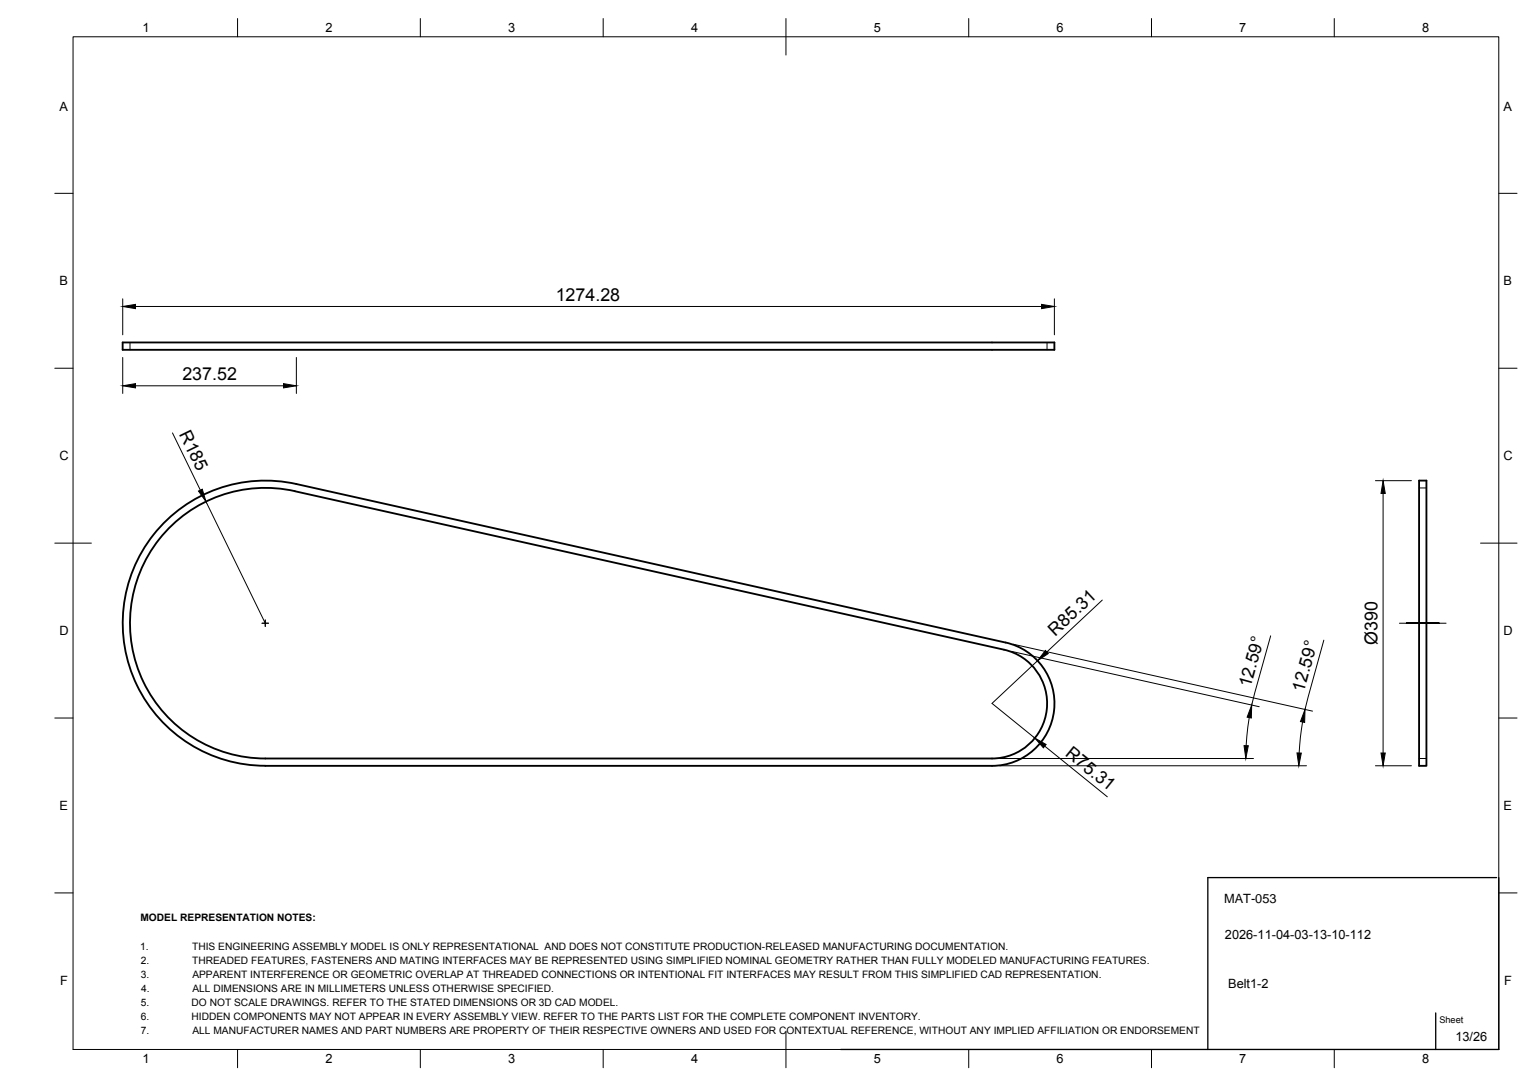
ISO-10303-21;
HEADER;
FILE_DESCRIPTION (('STEP AP214'),
    '1' );
FILE_NAME ('Belt1-2.step',
    '2026-10-10T03:43:58',
    ( '' ),
    ( '' ),
    'SwSTEP 2.0',
    'SolidWorks 2026',
    '' );
FILE_SCHEMA (( 'AUTOMOTIVE_DESIGN' ));
ENDSEC;

DATA;
#50=ORIENTED_EDGE ( 'NONE', *, *, #39637, .T. ) ;
#400=LINE ( 'NONE', #38040, #43022 ) ;
#483=ADVANCED_BREP_SHAPE_REPRESENTATION ( '', ( #63157, #66832 ), #16381 ) ;
#518=CIRCLE ( 'NONE', #7308, 85.31295361348101380 ) ;
#529=CARTESIAN_POINT ( 'NONE',  ( -737.6000277536880958, -694.2189502691660437, 10.00000000000000000 ) ) ;
#744=CARTESIAN_POINT ( 'NONE',  ( -783.0172411895269988, -622.0000000000060254, 0.000000000000000000 ) ) ;
#772=VERTEX_POINT ( 'NONE', #33537 ) ;
#796=CARTESIAN_POINT ( 'NONE',  ( -783.0172411895269988, -622.0000000000060254, 10.00000000000000000 ) ) ;
#912=( GEOMETRIC_REPRESENTATION_CONTEXT ( 3 ) GLOBAL_UNCERTAINTY_ASSIGNED_CONTEXT ( ( #67666 ) ) GLOBAL_UNIT_ASSIGNED_CONTEXT ( ( #33451, #27807, #26433 ) ) REPRESENTATION_CONTEXT ( 'NONE', 'WORKASPACE' ) );
#1644=ADVANCED_FACE ( 'NONE', ( #6203 ), #36842, .F. ) ;
#1813=ORIENTED_EDGE ( 'NONE', *, *, #39226, .T. ) ;
#1988=MECHANICAL_DESIGN_GEOMETRIC_PRESENTATION_REPRESENTATION('',(#14333),#912);
#2075=VECTOR ( 'NONE', #8776, 1000.000000000000227 ) ;
#2171=VERTEX_POINT ( 'NONE', #48575 ) ;
#2420=DIRECTION ( 'NONE',  ( 0.000000000000000000, 0.000000000000000000, 1.000000000000000000 ) ) ;
#2612=CARTESIAN_POINT ( 'NONE',  ( -137.3060924980642596, 138.4631249211268482, 10.00000000000000000 ) ) ;
#2773=ORIENTED_EDGE ( 'NONE', *, *, #39637, .F. ) ;
#3415=EDGE_CURVE ( 'NONE', #35337, #45327, #38767, .T. ) ;
#4052=EDGE_LOOP ( 'NONE', ( #25158, #36833, #15279, #17366 ) ) ;
#4364=VERTEX_POINT ( 'NONE', #44294 ) ;
#4376=CYLINDRICAL_SURFACE ( 'NONE', #64379, 185.0000000000000000 ) ;
#4633=CARTESIAN_POINT ( 'NONE',  ( -843.0889760620008246, -561.4220607509099636, 0.000000000000000000 ) ) ;
#4659=ORIENTED_EDGE ( 'NONE', *, *, #47648, .T. ) ;
#4808=DIRECTION ( 'NONE',  ( -1.000000000000000000, 0.000000000000000000, 0.000000000000000000 ) ) ;
#4817=EDGE_CURVE ( 'NONE', #23974, #44398, #13439, .T. ) ;
#5033=AXIS2_PLACEMENT_3D ( 'NONE', #67529, #67881, #9476 ) ;
#5314=SURFACE_SIDE_STYLE ('',( #53485 ) ) ;
#5328=COLOUR_RGB ( '',0.7921568627450980005, 0.8196078431372548767, 0.9333333333333333481 ) ;
#5721=CARTESIAN_POINT ( 'NONE',  ( -3.841371665203041630E-11, 0.000000000000000000, 10.00000000000000000 ) ) ;
#6203=FACE_OUTER_BOUND ( 'NONE', #4052, .T. ) ;
#6217=CARTESIAN_POINT ( 'NONE',  ( -783.0172411895269988, -622.0000000000060254, 10.00000000000000000 ) ) ;
#6235=AXIS2_PLACEMENT_3D ( 'NONE', #796, #54594, #6418 ) ;
#6350=FACE_OUTER_BOUND ( 'NONE', #25484, .T. ) ;
#6353=FILL_AREA_STYLE_COLOUR ( '', #5328 ) ;
#6418=DIRECTION ( 'NONE',  ( -1.000000000000000000, 0.000000000000000000, 0.000000000000000000 ) ) ;
#6578=EDGE_CURVE ( 'NONE', #4364, #56202, #63506, .T. ) ;
#6741=EDGE_CURVE ( 'NONE', #2171, #45327, #32909, .T. ) ;
#7096=AXIS2_PLACEMENT_3D ( 'NONE', #32587, #11821, #54011 ) ;
#7308=AXIS2_PLACEMENT_3D ( 'NONE', #55891, #7709, #49903 ) ;
#7350=FACE_OUTER_BOUND ( 'NONE', #64510, .T. ) ;
#7700=CYLINDRICAL_SURFACE ( 'NONE', #43072, 75.31295361348099959 ) ;
#7709=DIRECTION ( 'NONE',  ( 0.000000000000000000, 0.000000000000000000, 1.000000000000000000 ) ) ;
#7878=CARTESIAN_POINT ( 'NONE',  ( -3.841371665203041630E-11, 0.000000000000000000, 10.00000000000000000 ) ) ;
#7930=ORIENTED_EDGE ( 'NONE', *, *, #15029, .T. ) ;
#8319=DIRECTION ( 'NONE',  ( 1.000000000000000000, 0.000000000000000000, 0.000000000000000000 ) ) ;
#8395=DIRECTION ( 'NONE',  ( 1.000000000000000000, 0.000000000000000000, 0.000000000000000000 ) ) ;
#8400=CARTESIAN_POINT ( 'NONE',  ( -836.0476379851789943, -568.5227338237882577, 10.00000000000000000 ) ) ;
#8476=APPLICATION_CONTEXT ( 'automotive_design' ) ;
#8776=DIRECTION ( 'NONE',  ( 0.8465179929926601732, 0.5323601107705934199, 0.000000000000000000 ) ) ;
#8933=LINE ( 'NONE', #2612, #15335 ) ;
#8944=CARTESIAN_POINT ( 'NONE',  ( -783.0172411895269988, -622.0000000000060254, 10.00000000000000000 ) ) ;
#8997=VERTEX_POINT ( 'NONE', #19721 ) ;
#9476=DIRECTION ( 'NONE',  ( 1.000000000000000000, 0.000000000000000000, 0.000000000000000000 ) ) ;
#9556=CIRCLE ( 'NONE', #17419, 85.31295361348101380 ) ;
#10144=VECTOR ( 'NONE', #29624, 1000.000000000000000 ) ;
#10284=( LENGTH_UNIT ( ) NAMED_UNIT ( * ) SI_UNIT ( .MILLI., .METRE. ) );
#10312=DIRECTION ( 'NONE',  ( 1.000000000000000000, 0.000000000000000000, 0.000000000000000000 ) ) ;
#10925=EDGE_CURVE ( 'NONE', #23974, #31182, #64895, .T. ) ;
#10935=AXIS2_PLACEMENT_3D ( 'NONE', #21876, #32787, #32098 ) ;
#10980=CIRCLE ( 'NONE', #18831, 185.0000000000000000 ) ;
#11158=CARTESIAN_POINT ( 'NONE',  ( -836.0476379851789943, -568.5227338237882577, 10.00000000000000000 ) ) ;
#11197=VECTOR ( 'NONE', #34857, 1000.000000000000000 ) ;
#11821=DIRECTION ( 'NONE',  ( 0.000000000000000000, 0.000000000000000000, 1.000000000000000000 ) ) ;
#11932=CARTESIAN_POINT ( 'NONE',  ( 98.48662049252135375, -156.6058287036421461, 0.000000000000000000 ) ) ;
#11981=PRESENTATION_STYLE_ASSIGNMENT (( #60160 ) ) ;
#12058=APPLICATION_CONTEXT ( 'automotive_design' ) ;
#12469=ADVANCED_FACE ( 'NONE', ( #39879, #61340 ), #34625, .T. ) ;
#12980=CARTESIAN_POINT ( 'NONE',  ( -3.841371665203041630E-11, 0.000000000000000000, 10.00000000000000000 ) ) ;
#13197=CARTESIAN_POINT ( 'NONE',  ( -3.841371665203041630E-11, 0.000000000000000000, 10.00000000000000000 ) ) ;
#13360=CARTESIAN_POINT ( 'NONE',  ( -836.0476379851791080, -568.5227338237882577, 0.000000000000000000 ) ) ;
#13395=LINE ( 'NONE', #65470, #11197 ) ;
#13439=LINE ( 'NONE', #24692, #66682 ) ;
#13783=CIRCLE ( 'NONE', #16031, 75.31295361348099959 ) ;
#13838=DIRECTION ( 'NONE',  ( 1.000000000000000000, 0.000000000000000000, 0.000000000000000000 ) ) ;
#13899=CARTESIAN_POINT ( 'NONE',  ( -137.3060924980642596, 138.4631249211268482, 10.00000000000000000 ) ) ;
#14167=DIRECTION ( 'NONE',  ( 0.7041338076821838099, -0.7100673072878298520, 0.000000000000000000 ) ) ;
#14220=DIRECTION ( 'NONE',  ( -0.000000000000000000, -0.000000000000000000, -1.000000000000000000 ) ) ;
#14333=STYLED_ITEM ( 'NONE', ( #11981 ), #63157 ) ;
#14567=ORIENTED_EDGE ( 'NONE', *, *, #47164, .F. ) ;
#15029=EDGE_CURVE ( 'NONE', #51895, #35337, #62898, .T. ) ;
#15261=ORIENTED_EDGE ( 'NONE', *, *, #6578, .T. ) ;
#15279=ORIENTED_EDGE ( 'NONE', *, *, #15029, .F. ) ;
#15319=CARTESIAN_POINT ( 'NONE',  ( 98.48662049252135375, -156.6058287036421461, 10.00000000000000000 ) ) ;
#15335=VECTOR ( 'NONE', #18788, 1000.000000000000000 ) ;
#15471=ORIENTED_EDGE ( 'NONE', *, *, #37409, .F. ) ;
#15651=EDGE_CURVE ( 'NONE', #772, #4364, #61653, .T. ) ;
#15918=SHAPE_REPRESENTATION_RELATIONSHIP ( 'NONE' , 'NONE' ,  #46431, #483 ) ;
#15964=ORIENTED_EDGE ( 'NONE', *, *, #53374, .F. ) ;
#16014=ADVANCED_FACE ( 'NONE', ( #69170 ), #20998, .T. ) ;
#16031=AXIS2_PLACEMENT_3D ( 'NONE', #6217, #49820, #44190 ) ;
#16080=ORIENTED_EDGE ( 'NONE', *, *, #39226, .F. ) ;
#16381=( GEOMETRIC_REPRESENTATION_CONTEXT ( 3 ) GLOBAL_UNCERTAINTY_ASSIGNED_CONTEXT ( ( #49374 ) ) GLOBAL_UNIT_ASSIGNED_CONTEXT ( ( #10284, #38062, #27503 ) ) REPRESENTATION_CONTEXT ( 'NONE', 'WORKASPACE' ) );
#16466=ORIENTED_EDGE ( 'NONE', *, *, #59378, .F. ) ;
#16966=EDGE_CURVE ( 'NONE', #27319, #8997, #51411, .T. ) ;
#17366=ORIENTED_EDGE ( 'NONE', *, *, #60571, .T. ) ;
#17419=AXIS2_PLACEMENT_3D ( 'NONE', #744, #37673, #22198 ) ;
#17544=ORIENTED_EDGE ( 'NONE', *, *, #62686, .T. ) ;
#17563=LINE ( 'NONE', #65769, #42289 ) ;
#17823=LINE ( 'NONE', #61074, #45554 ) ;
#18035=ADVANCED_FACE ( 'NONE', ( #42232, #64032 ), #36959, .F. ) ;
#18131=LINE ( 'NONE', #35347, #47991 ) ;
#18788=DIRECTION ( 'NONE',  ( -0.000000000000000000, -0.000000000000000000, -1.000000000000000000 ) ) ;
#18820=ADVANCED_FACE ( 'NONE', ( #62405 ), #40948, .T. ) ;
#18831=AXIS2_PLACEMENT_3D ( 'NONE', #13197, #44497, #22692 ) ;
#18943=DIRECTION ( 'NONE',  ( -1.000000000000000000, 0.000000000000000000, 0.000000000000000000 ) ) ;
#19320=CLOSED_SHELL ( 'NONE', ( #40021, #16014, #12469, #18035, #28178, #1644, #18820, #20155, #25382, #30202, #67285, #52018 ) ) ;
#19721=CARTESIAN_POINT ( 'NONE',  ( -858.3301948030079984, -622.0000000000060254, 10.00000000000000000 ) ) ;
#20155=ADVANCED_FACE ( 'NONE', ( #6350 ), #27803, .F. ) ;
#20497=FACE_OUTER_BOUND ( 'NONE', #36320, .T. ) ;
#20652=CARTESIAN_POINT ( 'NONE',  ( -137.3060924980642596, 138.4631249211268482, 10.00000000000000000 ) ) ;
#20687=ORIENTED_EDGE ( 'NONE', *, *, #34883, .T. ) ;
#20771=CARTESIAN_POINT ( 'NONE',  ( -3.841371665203041630E-11, 0.000000000000000000, 0.000000000000000000 ) ) ;
#20998=CYLINDRICAL_SURFACE ( 'NONE', #65260, 85.31295361348101380 ) ;
#21143=ORIENTED_EDGE ( 'NONE', *, *, #47164, .T. ) ;
#21789=AXIS2_PLACEMENT_3D ( 'NONE', #25794, #31408, #13838 ) ;
#21825=FILL_AREA_STYLE ('',( #6353 ) ) ;
#21876=CARTESIAN_POINT ( 'NONE',  ( 98.48662049252141060, -156.6058287036421177, 10.00000000000000000 ) ) ;
#22198=DIRECTION ( 'NONE',  ( 1.000000000000000000, 0.000000000000000000, 0.000000000000000000 ) ) ;
#22214=DIRECTION ( 'NONE',  ( -0.000000000000000000, -0.000000000000000000, -1.000000000000000000 ) ) ;
#22249=FACE_OUTER_BOUND ( 'NONE', #61024, .T. ) ;
#22256=LINE ( 'NONE', #48960, #40432 ) ;
#22692=DIRECTION ( 'NONE',  ( 1.000000000000000000, 0.000000000000000000, 0.000000000000000000 ) ) ;
#23210=ORIENTED_EDGE ( 'NONE', *, *, #50303, .F. ) ;
#23231=ORIENTED_EDGE ( 'NONE', *, *, #6578, .F. ) ;
#23502=FACE_OUTER_BOUND ( 'NONE', #52077, .T. ) ;
#23851=CARTESIAN_POINT ( 'NONE',  ( -3.841371665203041630E-11, 0.000000000000000000, 10.00000000000000000 ) ) ;
#23972=CIRCLE ( 'NONE', #7096, 185.0000000000000000 ) ;
#23974=VERTEX_POINT ( 'NONE', #29767 ) ;
#24090=DIRECTION ( 'NONE',  ( -1.000000000000000000, 0.000000000000000000, 0.000000000000000000 ) ) ;
#24259=CARTESIAN_POINT ( 'NONE',  ( -737.6000277536880958, -694.2189502691659300, 10.00000000000000000 ) ) ;
#24630=DIRECTION ( 'NONE',  ( -0.8465179929926601732, -0.5323601107705934199, 0.000000000000000000 ) ) ;
#24692=CARTESIAN_POINT ( 'NONE',  ( -868.3301948030079984, -622.0000000000060254, 10.00000000000000000 ) ) ;
#24825=EDGE_LOOP ( 'NONE', ( #4659, #54553, #25083, #1813, #17544 ) ) ;
#25083=ORIENTED_EDGE ( 'NONE', *, *, #59378, .T. ) ;
#25158=ORIENTED_EDGE ( 'NONE', *, *, #6741, .T. ) ;
#25382=ADVANCED_FACE ( 'NONE', ( #22249 ), #65162, .F. ) ;
#25383=PRODUCT ( 'Belt1-2', 'Belt1-2', '', ( #62124 ) ) ;
#25484=EDGE_LOOP ( 'NONE', ( #39915, #52107, #61469, #50 ) ) ;
#25591=AXIS2_PLACEMENT_3D ( 'NONE', #7878, #29328, #34144 ) ;
#25794=CARTESIAN_POINT ( 'NONE',  ( -3.841371665203041630E-11, 0.000000000000000000, 0.000000000000000000 ) ) ;
#26049=AXIS2_PLACEMENT_3D ( 'NONE', #20771, #32027, #65071 ) ;
#26141=EDGE_CURVE ( 'NONE', #45146, #51895, #60214, .T. ) ;
#26226=SHAPE_DEFINITION_REPRESENTATION ( #30409, #46431 ) ;
#26433=( NAMED_UNIT ( * ) SI_UNIT ( $, .STERADIAN. ) SOLID_ANGLE_UNIT ( ) );
#26631=DIRECTION ( 'NONE',  ( 0.7041338076821838099, -0.7100673072878299630, 0.000000000000000000 ) ) ;
#26818=EDGE_CURVE ( 'NONE', #44398, #46298, #9556, .T. ) ;
#27319=VERTEX_POINT ( 'NONE', #28624 ) ;
#27327=VECTOR ( 'NONE', #54051, 1000.000000000000000 ) ;
#27445=VERTEX_POINT ( 'NONE', #57433 ) ;
#27503=( NAMED_UNIT ( * ) SI_UNIT ( $, .STERADIAN. ) SOLID_ANGLE_UNIT ( ) );
#27615=AXIS2_PLACEMENT_3D ( 'NONE', #12980, #39355, #18943 ) ;
#27632=CARTESIAN_POINT ( 'NONE',  ( -137.3060924980642596, 138.4631249211268482, 0.000000000000000000 ) ) ;
#27803=PLANE ( 'NONE',  #28332 ) ;
#27807=( NAMED_UNIT ( * ) PLANE_ANGLE_UNIT ( ) SI_UNIT ( $, .RADIAN. ) );
#28178=ADVANCED_FACE ( 'NONE', ( #51648 ), #45320, .T. ) ;
#28332=AXIS2_PLACEMENT_3D ( 'NONE', #49243, #29894, #24630 ) ;
#28472=ORIENTED_EDGE ( 'NONE', *, *, #6741, .F. ) ;
#28624=CARTESIAN_POINT ( 'NONE',  ( -836.0476379851789943, -568.5227338237882577, 10.00000000000000000 ) ) ;
#29153=EDGE_CURVE ( 'NONE', #45146, #58415, #17563, .T. ) ;
#29328=DIRECTION ( 'NONE',  ( 0.000000000000000000, 0.000000000000000000, 1.000000000000000000 ) ) ;
#29344=ORIENTED_EDGE ( 'NONE', *, *, #69178, .T. ) ;
#29624=DIRECTION ( 'NONE',  ( -0.000000000000000000, -0.000000000000000000, -1.000000000000000000 ) ) ;
#29767=CARTESIAN_POINT ( 'NONE',  ( -868.3301948030079984, -622.0000000000060254, 10.00000000000000000 ) ) ;
#29894=DIRECTION ( 'NONE',  ( -0.5323601107705935309, 0.8465179929926602842, 0.000000000000000000 ) ) ;
#30201=DIRECTION ( 'NONE',  ( -0.7100673072878298520, -0.7041338076821836989, 0.000000000000000000 ) ) ;
#30202=ADVANCED_FACE ( 'NONE', ( #20497 ), #59160, .T. ) ;
#30409=PRODUCT_DEFINITION_SHAPE ( 'NONE', 'NONE',  #54682 ) ;
#30539=CARTESIAN_POINT ( 'NONE',  ( -137.3060924980642596, 138.4631249211268482, 10.00000000000000000 ) ) ;
#31087=CARTESIAN_POINT ( 'NONE',  ( -742.9236288613935812, -685.7537703392392814, 10.00000000000000000 ) ) ;
#31182=VERTEX_POINT ( 'NONE', #529 ) ;
#31408=DIRECTION ( 'NONE',  ( 0.000000000000000000, 0.000000000000000000, 1.000000000000000000 ) ) ;
#31420=ORIENTED_EDGE ( 'NONE', *, *, #16966, .T. ) ;
#32016=VECTOR ( 'NONE', #57545, 1000.000000000000000 ) ;
#32027=DIRECTION ( 'NONE',  ( 0.000000000000000000, 0.000000000000000000, 1.000000000000000000 ) ) ;
#32098=DIRECTION ( 'NONE',  ( -0.8465179929926601732, -0.5323601107705934199, 0.000000000000000000 ) ) ;
#32587=CARTESIAN_POINT ( 'NONE',  ( -3.841371665203041630E-11, 0.000000000000000000, 0.000000000000000000 ) ) ;
#32648=ORIENTED_EDGE ( 'NONE', *, *, #56944, .F. ) ;
#32695=DIRECTION ( 'NONE',  ( -0.000000000000000000, -0.000000000000000000, -1.000000000000000000 ) ) ;
#32702=ORIENTED_EDGE ( 'NONE', *, *, #69229, .T. ) ;
#32787=DIRECTION ( 'NONE',  ( -0.5323601107705935309, 0.8465179929926602842, 0.000000000000000000 ) ) ;
#32812=ORIENTED_EDGE ( 'NONE', *, *, #50303, .T. ) ;
#32909=LINE ( 'NONE', #27632, #33121 ) ;
#32935=DIRECTION ( 'NONE',  ( 0.7100673072878298520, 0.7041338076821836989, 0.000000000000000000 ) ) ;
#33121=VECTOR ( 'NONE', #49069, 1000.000000000000114 ) ;
#33204=EDGE_LOOP ( 'NONE', ( #49834, #56468, #51894, #56685, #28472 ) ) ;
#33451=( LENGTH_UNIT ( ) NAMED_UNIT ( * ) SI_UNIT ( .MILLI., .METRE. ) );
#33537=CARTESIAN_POINT ( 'NONE',  ( -742.9236288613935812, -685.7537703392392814, 10.00000000000000000 ) ) ;
#34133=ORIENTED_EDGE ( 'NONE', *, *, #69229, .F. ) ;
#34144=DIRECTION ( 'NONE',  ( 1.000000000000000000, 0.000000000000000000, -0.000000000000000000 ) ) ;
#34194=DIRECTION ( 'NONE',  ( -0.000000000000000000, -0.000000000000000000, -1.000000000000000000 ) ) ;
#34218=ORIENTED_EDGE ( 'NONE', *, *, #10925, .T. ) ;
#34226=VECTOR ( 'NONE', #40058, 1000.000000000000227 ) ;
#34568=ORIENTED_EDGE ( 'NONE', *, *, #4817, .F. ) ;
#34584=CARTESIAN_POINT ( 'NONE',  ( -130.2647544212423725, 131.3624518482485541, 10.00000000000000000 ) ) ;
#34625=PLANE ( 'NONE',  #25591 ) ;
#34857=DIRECTION ( 'NONE',  ( -0.000000000000000000, -0.000000000000000000, -1.000000000000000000 ) ) ;
#34883=EDGE_CURVE ( 'NONE', #8997, #64350, #13395, .T. ) ;
#34930=CARTESIAN_POINT ( 'NONE',  ( 98.48662049252141060, -156.6058287036421177, 10.00000000000000000 ) ) ;
#35109=DIRECTION ( 'NONE',  ( -0.000000000000000000, -0.000000000000000000, -1.000000000000000000 ) ) ;
#35173=CARTESIAN_POINT ( 'NONE',  ( -868.3301948030079984, -622.0000000000060254, 0.000000000000000000 ) ) ;
#35276=CARTESIAN_POINT ( 'NONE',  ( -836.0476379851789943, -568.5227338237882577, 10.00000000000000000 ) ) ;
#35337=VERTEX_POINT ( 'NONE', #68499 ) ;
#35347=CARTESIAN_POINT ( 'NONE',  ( -836.0476379851789943, -568.5227338237882577, 0.000000000000000000 ) ) ;
#36292=EDGE_LOOP ( 'NONE', ( #42354, #7930, #21143, #34218, #55338 ) ) ;
#36320=EDGE_LOOP ( 'NONE', ( #16466, #15471, #55287, #15261 ) ) ;
#36486=CARTESIAN_POINT ( 'NONE',  ( -783.0172411895269988, -622.0000000000060254, 10.00000000000000000 ) ) ;
#36487=DIRECTION ( 'NONE',  ( 1.000000000000000000, 0.000000000000000000, 0.000000000000000000 ) ) ;
#36833=ORIENTED_EDGE ( 'NONE', *, *, #3415, .F. ) ;
#36842=PLANE ( 'NONE',  #58757 ) ;
#36959=PLANE ( 'NONE',  #26049 ) ;
#37409=EDGE_CURVE ( 'NONE', #772, #54998, #53195, .T. ) ;
#37673=DIRECTION ( 'NONE',  ( 0.000000000000000000, 0.000000000000000000, 1.000000000000000000 ) ) ;
#38040=CARTESIAN_POINT ( 'NONE',  ( -737.6000277536880958, -694.2189502691660437, 10.00000000000000000 ) ) ;
#38062=( NAMED_UNIT ( * ) PLANE_ANGLE_UNIT ( ) SI_UNIT ( $, .RADIAN. ) );
#38767=LINE ( 'NONE', #54216, #47613 ) ;
#38942=DIRECTION ( 'NONE',  ( 0.000000000000000000, 0.000000000000000000, 1.000000000000000000 ) ) ;
#39033=AXIS2_PLACEMENT_3D ( 'NONE', #42219, #38942, #49817 ) ;
#39226=EDGE_CURVE ( 'NONE', #56202, #39748, #23972, .T. ) ;
#39280=DIRECTION ( 'NONE',  ( 0.8465179929926601732, 0.5323601107705934199, -0.000000000000000000 ) ) ;
#39355=DIRECTION ( 'NONE',  ( -0.000000000000000000, -0.000000000000000000, -1.000000000000000000 ) ) ;
#39623=DIRECTION ( 'NONE',  ( 1.000000000000000000, 0.000000000000000000, 0.000000000000000000 ) ) ;
#39637=EDGE_CURVE ( 'NONE', #31182, #46298, #400, .T. ) ;
#39711=LINE ( 'NONE', #8400, #34226 ) ;
#39748=VERTEX_POINT ( 'NONE', #61917 ) ;
#39879=FACE_OUTER_BOUND ( 'NONE', #36292, .T. ) ;
#39915=ORIENTED_EDGE ( 'NONE', *, *, #65294, .T. ) ;
#40021=ADVANCED_FACE ( 'NONE', ( #7350 ), #7700, .F. ) ;
#40058=DIRECTION ( 'NONE',  ( -0.7100673072878298520, -0.7041338076821838099, -0.000000000000000000 ) ) ;
#40277=DIRECTION ( 'NONE',  ( -0.7100673072878298520, -0.7041338076821838099, -0.000000000000000000 ) ) ;
#40432=VECTOR ( 'NONE', #65168, 1000.000000000000227 ) ;
#40505=CARTESIAN_POINT ( 'NONE',  ( -742.9236288613935812, -685.7537703392392814, 0.000000000000000000 ) ) ;
#40539=DIRECTION ( 'NONE',  ( 0.8465179929926601732, 0.5323601107705934199, -0.000000000000000000 ) ) ;
#40645=AXIS2_PLACEMENT_3D ( 'NONE', #35276, #14167, #45476 ) ;
#40648=EDGE_CURVE ( 'NONE', #58415, #2171, #53214, .T. ) ;
#40948=CYLINDRICAL_SURFACE ( 'NONE', #65298, 85.31295361348101380 ) ;
#40955=ORIENTED_EDGE ( 'NONE', *, *, #10925, .F. ) ;
#40990=AXIS2_PLACEMENT_3D ( 'NONE', #5721, #64827, #10312 ) ;
#41665=VECTOR ( 'NONE', #40539, 1000.000000000000227 ) ;
#42219=CARTESIAN_POINT ( 'NONE',  ( -783.0172411895269988, -622.0000000000060254, 0.000000000000000000 ) ) ;
#42232=FACE_OUTER_BOUND ( 'NONE', #33204, .T. ) ;
#42289=VECTOR ( 'NONE', #32695, 1000.000000000000000 ) ;
#42354=ORIENTED_EDGE ( 'NONE', *, *, #26141, .T. ) ;
#42621=ORIENTED_EDGE ( 'NONE', *, *, #4817, .T. ) ;
#43022=VECTOR ( 'NONE', #22214, 1000.000000000000000 ) ;
#43072=AXIS2_PLACEMENT_3D ( 'NONE', #46347, #35109, #61155 ) ;
#43231=CIRCLE ( 'NONE', #5033, 75.31295361348099959 ) ;
#44190=DIRECTION ( 'NONE',  ( 1.000000000000000000, 0.000000000000000000, 0.000000000000000000 ) ) ;
#44249=ORIENTED_EDGE ( 'NONE', *, *, #26818, .T. ) ;
#44294=CARTESIAN_POINT ( 'NONE',  ( 98.48662049252135375, -156.6058287036421461, 10.00000000000000000 ) ) ;
#44398=VERTEX_POINT ( 'NONE', #35173 ) ;
#44428=ORIENTED_EDGE ( 'NONE', *, *, #54193, .F. ) ;
#44497=DIRECTION ( 'NONE',  ( 0.000000000000000000, 0.000000000000000000, 1.000000000000000000 ) ) ;
#44558=DIRECTION ( 'NONE',  ( 0.000000000000000000, 0.000000000000000000, 1.000000000000000000 ) ) ;
#44641=ORIENTED_EDGE ( 'NONE', *, *, #53374, .T. ) ;
#45146=VERTEX_POINT ( 'NONE', #60617 ) ;
#45289=DIRECTION ( 'NONE',  ( -0.000000000000000000, -0.000000000000000000, -1.000000000000000000 ) ) ;
#45320=CYLINDRICAL_SURFACE ( 'NONE', #27615, 195.0000000000000000 ) ;
#45327=VERTEX_POINT ( 'NONE', #4633 ) ;
#45476=DIRECTION ( 'NONE',  ( 0.7100673072878298520, 0.7041338076821838099, 0.000000000000000000 ) ) ;
#45554=VECTOR ( 'NONE', #39280, 1000.000000000000227 ) ;
#45638=ORIENTED_EDGE ( 'NONE', *, *, #66493, .T. ) ;
#45985=ORIENTED_EDGE ( 'NONE', *, *, #15651, .F. ) ;
#46298=VERTEX_POINT ( 'NONE', #63056 ) ;
#46347=CARTESIAN_POINT ( 'NONE',  ( -783.0172411895269988, -622.0000000000060254, 10.00000000000000000 ) ) ;
#46431=SHAPE_REPRESENTATION ( 'Belt1-2', ( #66832 ), #16381 ) ;
#46647=EDGE_LOOP ( 'NONE', ( #40955, #42621, #44249, #2773 ) ) ;
#47123=ORIENTED_EDGE ( 'NONE', *, *, #16966, .F. ) ;
#47164=EDGE_CURVE ( 'NONE', #35337, #23974, #51384, .T. ) ;
#47240=DIRECTION ( 'NONE',  ( -0.000000000000000000, -0.000000000000000000, -1.000000000000000000 ) ) ;
#47403=LINE ( 'NONE', #11158, #27327 ) ;
#47613=VECTOR ( 'NONE', #34194, 1000.000000000000000 ) ;
#47648=EDGE_CURVE ( 'NONE', #49666, #64350, #53609, .T. ) ;
#47736=ORIENTED_EDGE ( 'NONE', *, *, #34883, .F. ) ;
#47767=EDGE_LOOP ( 'NONE', ( #45985, #15964, #47123, #34133, #23210 ) ) ;
#47984=AXIS2_PLACEMENT_3D ( 'NONE', #59664, #55440, #39623 ) ;
#47991=VECTOR ( 'NONE', #40277, 1000.000000000000227 ) ;
#48058=CARTESIAN_POINT ( 'NONE',  ( -783.0172411895269988, -622.0000000000060254, 10.00000000000000000 ) ) ;
#48129=EDGE_LOOP ( 'NONE', ( #34568, #14567, #50181, #29344 ) ) ;
#48479=EDGE_CURVE ( 'NONE', #31182, #45146, #63265, .T. ) ;
#48575=CARTESIAN_POINT ( 'NONE',  ( -137.3060924980642596, 138.4631249211268482, 0.000000000000000000 ) ) ;
#48960=CARTESIAN_POINT ( 'NONE',  ( -737.6000277536880958, -694.2189502691659300, 0.000000000000000000 ) ) ;
#49069=DIRECTION ( 'NONE',  ( -0.7100673072878298520, -0.7041338076821836989, 0.000000000000000000 ) ) ;
#49243=CARTESIAN_POINT ( 'NONE',  ( -737.6000277536880958, -694.2189502691659300, 10.00000000000000000 ) ) ;
#49254=CARTESIAN_POINT ( 'NONE',  ( 103.8102216002272939, -165.0710086335687379, 0.000000000000000000 ) ) ;
#49374=UNCERTAINTY_MEASURE_WITH_UNIT (LENGTH_MEASURE( 1.000000000000000082E-05 ), #10284, 'distance_accuracy_value', 'NONE');
#49666=VERTEX_POINT ( 'NONE', #13360 ) ;
#49817=DIRECTION ( 'NONE',  ( 1.000000000000000000, 0.000000000000000000, 0.000000000000000000 ) ) ;
#49820=DIRECTION ( 'NONE',  ( 0.000000000000000000, 0.000000000000000000, 1.000000000000000000 ) ) ;
#49834=ORIENTED_EDGE ( 'NONE', *, *, #40648, .F. ) ;
#49903=DIRECTION ( 'NONE',  ( 1.000000000000000000, 0.000000000000000000, 0.000000000000000000 ) ) ;
#50181=ORIENTED_EDGE ( 'NONE', *, *, #3415, .T. ) ;
#50303=EDGE_CURVE ( 'NONE', #4364, #27445, #10980, .T. ) ;
#50530=CARTESIAN_POINT ( 'NONE',  ( 0.000000000000000000, 0.000000000000000000, 0.000000000000000000 ) ) ;
#50600=CARTESIAN_POINT ( 'NONE',  ( -783.0172411895269988, -622.0000000000060254, 10.00000000000000000 ) ) ;
#50732=LINE ( 'NONE', #34584, #10144 ) ;
#51072=DIRECTION ( 'NONE',  ( -0.000000000000000000, -0.000000000000000000, -1.000000000000000000 ) ) ;
#51384=CIRCLE ( 'NONE', #47984, 85.31295361348101380 ) ;
#51411=CIRCLE ( 'NONE', #62799, 75.31295361348099959 ) ;
#51648=FACE_OUTER_BOUND ( 'NONE', #59751, .T. ) ;
#51894=ORIENTED_EDGE ( 'NONE', *, *, #26818, .F. ) ;
#51895=VERTEX_POINT ( 'NONE', #13899 ) ;
#51924=ORIENTED_EDGE ( 'NONE', *, *, #66493, .F. ) ;
#52018=ADVANCED_FACE ( 'NONE', ( #60963 ), #66957, .T. ) ;
#52077=EDGE_LOOP ( 'NONE', ( #16080, #23231, #32812, #45638 ) ) ;
#52107=ORIENTED_EDGE ( 'NONE', *, *, #29153, .F. ) ;
#52190=ORIENTED_EDGE ( 'NONE', *, *, #60571, .F. ) ;
#52839=PRODUCT_DEFINITION_CONTEXT ( 'detailed design', #12058, 'design' ) ;
#53127=EDGE_LOOP ( 'NONE', ( #60139, #51924, #32702, #65204 ) ) ;
#53195=LINE ( 'NONE', #31087, #64230 ) ;
#53214=CIRCLE ( 'NONE', #21789, 195.0000000000000000 ) ;
#53374=EDGE_CURVE ( 'NONE', #8997, #772, #13783, .T. ) ;
#53485=SURFACE_STYLE_FILL_AREA ( #21825 ) ;
#53609=CIRCLE ( 'NONE', #39033, 75.31295361348099959 ) ;
#54011=DIRECTION ( 'NONE',  ( 1.000000000000000000, 0.000000000000000000, 0.000000000000000000 ) ) ;
#54051=DIRECTION ( 'NONE',  ( -0.000000000000000000, -0.000000000000000000, -1.000000000000000000 ) ) ;
#54193=EDGE_CURVE ( 'NONE', #27319, #49666, #47403, .T. ) ;
#54216=CARTESIAN_POINT ( 'NONE',  ( -843.0889760620008246, -561.4220607509099636, 10.00000000000000000 ) ) ;
#54553=ORIENTED_EDGE ( 'NONE', *, *, #56944, .T. ) ;
#54594=DIRECTION ( 'NONE',  ( -0.000000000000000000, -0.000000000000000000, -1.000000000000000000 ) ) ;
#54682=PRODUCT_DEFINITION ( 'UNKNOWN', '', #69200, #52839 ) ;
#54998=VERTEX_POINT ( 'NONE', #40505 ) ;
#55287=ORIENTED_EDGE ( 'NONE', *, *, #15651, .T. ) ;
#55338=ORIENTED_EDGE ( 'NONE', *, *, #48479, .T. ) ;
#55440=DIRECTION ( 'NONE',  ( 0.000000000000000000, 0.000000000000000000, 1.000000000000000000 ) ) ;
#55891=CARTESIAN_POINT ( 'NONE',  ( -783.0172411895269988, -622.0000000000060254, 0.000000000000000000 ) ) ;
#56187=ORIENTED_EDGE ( 'NONE', *, *, #26141, .F. ) ;
#56202=VERTEX_POINT ( 'NONE', #11932 ) ;
#56468=ORIENTED_EDGE ( 'NONE', *, *, #65294, .F. ) ;
#56685=ORIENTED_EDGE ( 'NONE', *, *, #69178, .F. ) ;
#56944=EDGE_CURVE ( 'NONE', #64350, #54998, #43231, .T. ) ;
#57161=ORIENTED_EDGE ( 'NONE', *, *, #37409, .T. ) ;
#57384=VECTOR ( 'NONE', #30201, 1000.000000000000114 ) ;
#57433=CARTESIAN_POINT ( 'NONE',  ( -130.2647544212423725, 131.3624518482487247, 10.00000000000000000 ) ) ;
#57545=DIRECTION ( 'NONE',  ( -0.000000000000000000, -0.000000000000000000, -1.000000000000000000 ) ) ;
#57838=DIRECTION ( 'NONE',  ( -1.000000000000000000, 0.000000000000000000, 0.000000000000000000 ) ) ;
#58415=VERTEX_POINT ( 'NONE', #49254 ) ;
#58757=AXIS2_PLACEMENT_3D ( 'NONE', #20652, #26631, #32935 ) ;
#59160=PLANE ( 'NONE',  #10935 ) ;
#59378=EDGE_CURVE ( 'NONE', #54998, #56202, #17823, .T. ) ;
#59664=CARTESIAN_POINT ( 'NONE',  ( -783.0172411895269988, -622.0000000000060254, 10.00000000000000000 ) ) ;
#59751=EDGE_LOOP ( 'NONE', ( #67526, #52190, #56187, #67505 ) ) ;
#60139=ORIENTED_EDGE ( 'NONE', *, *, #62686, .F. ) ;
#60160=SURFACE_STYLE_USAGE ( .BOTH. , #5314 ) ;
#60214=CIRCLE ( 'NONE', #40990, 195.0000000000000000 ) ;
#60571=EDGE_CURVE ( 'NONE', #51895, #2171, #8933, .T. ) ;
#60617=CARTESIAN_POINT ( 'NONE',  ( 103.8102216002272939, -165.0710086335687379, 10.00000000000000000 ) ) ;
#60963=FACE_OUTER_BOUND ( 'NONE', #53127, .T. ) ;
#61024=EDGE_LOOP ( 'NONE', ( #47736, #44641, #57161, #32648 ) ) ;
#61074=CARTESIAN_POINT ( 'NONE',  ( 98.48662049252141060, -156.6058287036421177, 0.000000000000000000 ) ) ;
#61155=DIRECTION ( 'NONE',  ( -1.000000000000000000, 0.000000000000000000, 0.000000000000000000 ) ) ;
#61340=FACE_BOUND ( 'NONE', #47767, .T. ) ;
#61469=ORIENTED_EDGE ( 'NONE', *, *, #48479, .F. ) ;
#61653=LINE ( 'NONE', #34930, #41665 ) ;
#61677=ORIENTED_EDGE ( 'NONE', *, *, #47648, .F. ) ;
#61917=CARTESIAN_POINT ( 'NONE',  ( -130.2647544212423725, 131.3624518482485541, 0.000000000000000000 ) ) ;
#62124=PRODUCT_CONTEXT ( 'NONE', #8476, 'mechanical' ) ;
#62405=FACE_OUTER_BOUND ( 'NONE', #48129, .T. ) ;
#62686=EDGE_CURVE ( 'NONE', #39748, #49666, #18131, .T. ) ;
#62799=AXIS2_PLACEMENT_3D ( 'NONE', #50600, #2420, #8395 ) ;
#62898=LINE ( 'NONE', #30539, #57384 ) ;
#63056=CARTESIAN_POINT ( 'NONE',  ( -737.6000277536880958, -694.2189502691660437, 0.000000000000000000 ) ) ;
#63157=MANIFOLD_SOLID_BREP ( 'Boss-Extrude1', #19320 ) ;
#63220=DIRECTION ( 'NONE',  ( -0.000000000000000000, -0.000000000000000000, -1.000000000000000000 ) ) ;
#63265=LINE ( 'NONE', #24259, #2075 ) ;
#63506=LINE ( 'NONE', #15319, #32016 ) ;
#64032=FACE_BOUND ( 'NONE', #24825, .T. ) ;
#64230=VECTOR ( 'NONE', #47240, 1000.000000000000000 ) ;
#64350=VERTEX_POINT ( 'NONE', #64364 ) ;
#64364=CARTESIAN_POINT ( 'NONE',  ( -858.3301948030079984, -622.0000000000060254, 0.000000000000000000 ) ) ;
#64379=AXIS2_PLACEMENT_3D ( 'NONE', #23851, #45289, #57838 ) ;
#64510=EDGE_LOOP ( 'NONE', ( #31420, #20687, #61677, #44428 ) ) ;
#64827=DIRECTION ( 'NONE',  ( 0.000000000000000000, 0.000000000000000000, 1.000000000000000000 ) ) ;
#64895=CIRCLE ( 'NONE', #68275, 85.31295361348101380 ) ;
#65071=DIRECTION ( 'NONE',  ( 1.000000000000000000, 0.000000000000000000, -0.000000000000000000 ) ) ;
#65162=CYLINDRICAL_SURFACE ( 'NONE', #6235, 75.31295361348099959 ) ;
#65168=DIRECTION ( 'NONE',  ( 0.8465179929926601732, 0.5323601107705934199, 0.000000000000000000 ) ) ;
#65204=ORIENTED_EDGE ( 'NONE', *, *, #54193, .T. ) ;
#65260=AXIS2_PLACEMENT_3D ( 'NONE', #36486, #63220, #4808 ) ;
#65294=EDGE_CURVE ( 'NONE', #46298, #58415, #22256, .T. ) ;
#65298=AXIS2_PLACEMENT_3D ( 'NONE', #8944, #14220, #24090 ) ;
#65470=CARTESIAN_POINT ( 'NONE',  ( -858.3301948030079984, -622.0000000000060254, 10.00000000000000000 ) ) ;
#65769=CARTESIAN_POINT ( 'NONE',  ( 103.8102216002272939, -165.0710086335687379, 10.00000000000000000 ) ) ;
#66493=EDGE_CURVE ( 'NONE', #27445, #39748, #50732, .T. ) ;
#66682=VECTOR ( 'NONE', #51072, 1000.000000000000000 ) ;
#66832=AXIS2_PLACEMENT_3D ( 'NONE', #50530, #44558, #8319 ) ;
#66957=PLANE ( 'NONE',  #40645 ) ;
#67285=ADVANCED_FACE ( 'NONE', ( #23502 ), #4376, .F. ) ;
#67505=ORIENTED_EDGE ( 'NONE', *, *, #29153, .T. ) ;
#67526=ORIENTED_EDGE ( 'NONE', *, *, #40648, .T. ) ;
#67529=CARTESIAN_POINT ( 'NONE',  ( -783.0172411895269988, -622.0000000000060254, 0.000000000000000000 ) ) ;
#67666=UNCERTAINTY_MEASURE_WITH_UNIT (LENGTH_MEASURE( 1.000000000000000082E-05 ), #33451, 'distance_accuracy_value', 'NONE');
#67881=DIRECTION ( 'NONE',  ( 0.000000000000000000, 0.000000000000000000, 1.000000000000000000 ) ) ;
#68275=AXIS2_PLACEMENT_3D ( 'NONE', #48058, #69512, #36487 ) ;
#68499=CARTESIAN_POINT ( 'NONE',  ( -843.0889760620008246, -561.4220607509099636, 10.00000000000000000 ) ) ;
#69170=FACE_OUTER_BOUND ( 'NONE', #46647, .T. ) ;
#69178=EDGE_CURVE ( 'NONE', #45327, #44398, #518, .T. ) ;
#69200=PRODUCT_DEFINITION_FORMATION_WITH_SPECIFIED_SOURCE ( 'ANY', '', #25383, .NOT_KNOWN. ) ;
#69229=EDGE_CURVE ( 'NONE', #27445, #27319, #39711, .T. ) ;
#69512=DIRECTION ( 'NONE',  ( 0.000000000000000000, 0.000000000000000000, 1.000000000000000000 ) ) ;
ENDSEC;
END-ISO-10303-21;
